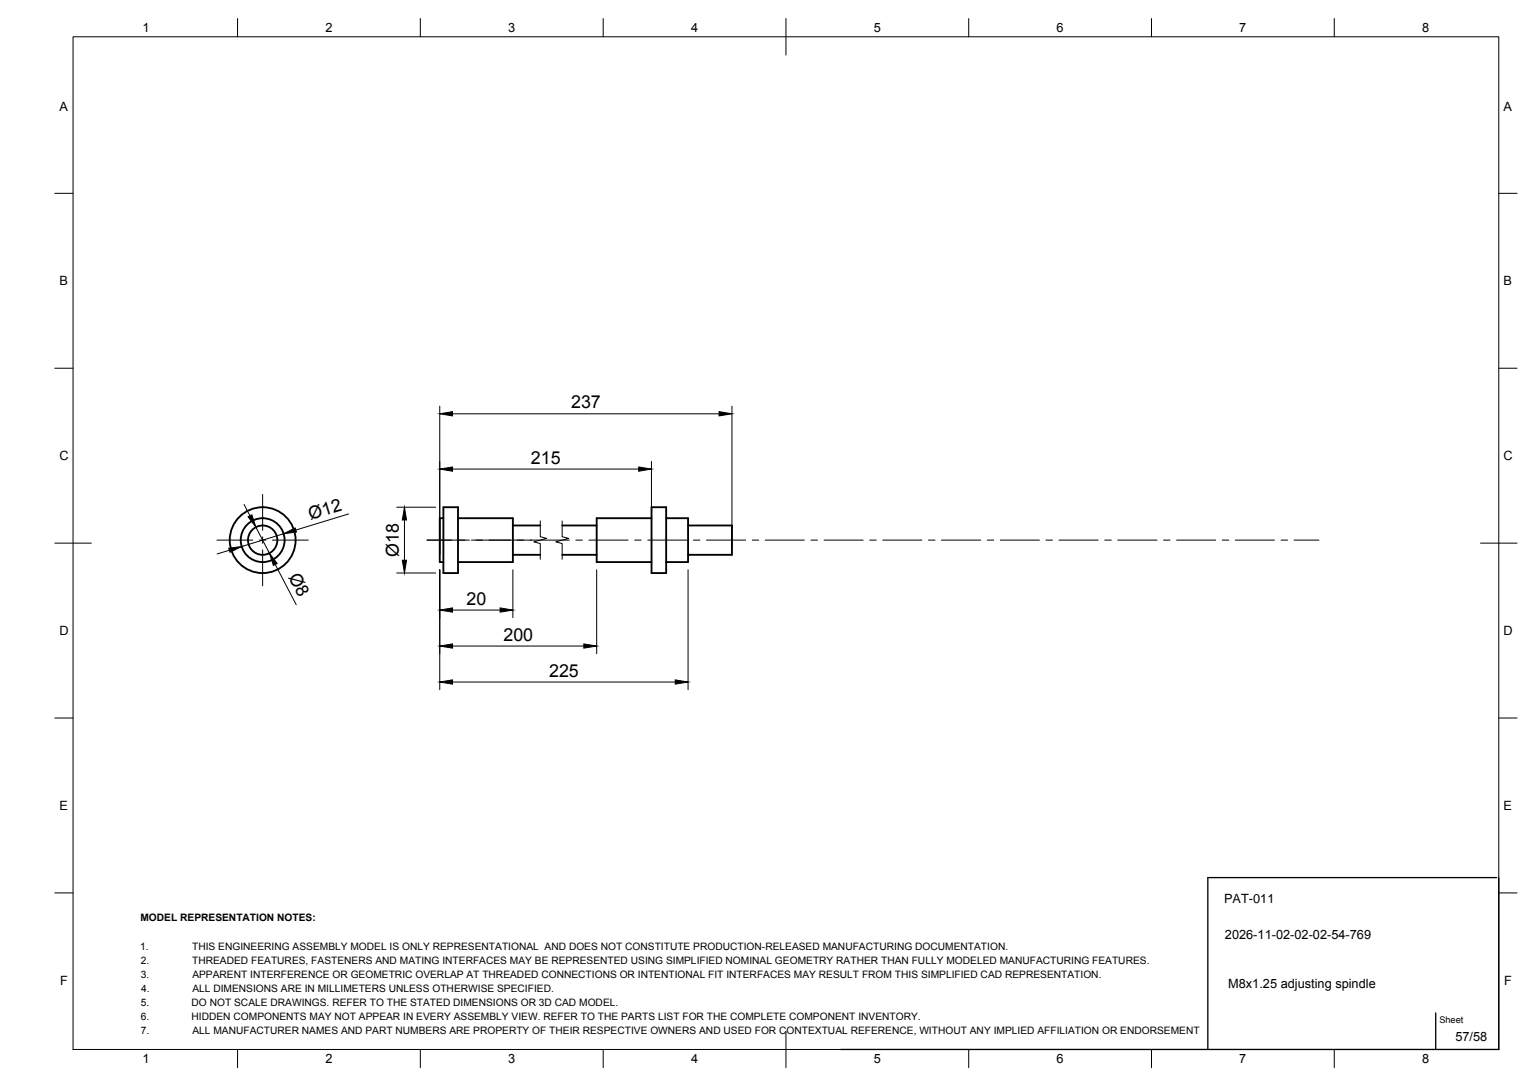
ISO-10303-21;
HEADER;
/* Generated by software containing ST-Developer
 * from STEP Tools, Inc. (www.steptools.com) 
 */

FILE_DESCRIPTION(
/* description */ ('Belt tension measurement rig'),
/* implementation_level */ '2;1');

FILE_NAME(
/* name */ 'M8x1.25 adjusting spindle.step',
/* time_stamp */ '2026-10-28T03:24:44-07:00',
/* author */ (''),
/* organization */ (''),
/* preprocessor_version */ 'ST-DEVELOPER v20.2',
/* originating_system */ 'Autodesk Translation Framework v15.17.0.0',
/* authorisation */ '');

FILE_SCHEMA (('AUTOMOTIVE_DESIGN { 1 0 10303 214 3 1 1 }'));
ENDSEC;

DATA;
#10=MECHANICAL_DESIGN_GEOMETRIC_PRESENTATION_REPRESENTATION('',(#759),#23587);
#634=SHAPE_REPRESENTATION_RELATIONSHIP('SRR','None',#23886,#689);
#689=ADVANCED_BREP_SHAPE_REPRESENTATION('',(#826),#23584);
#759=STYLED_ITEM('',(#24197),#826);
#826=MANIFOLD_SOLID_BREP('Body1',#12267);
#1027=FACE_BOUND('',#2925,.T.);
#1028=FACE_BOUND('',#2927,.T.);
#1029=FACE_BOUND('',#2931,.T.);
#1030=FACE_BOUND('',#2933,.T.);
#1031=FACE_BOUND('',#2937,.T.);
#1032=FACE_BOUND('',#2940,.T.);
#1033=FACE_BOUND('',#2945,.T.);
#1330=PLANE('',#14418);
#1331=PLANE('',#14419);
#1332=PLANE('',#14422);
#1333=PLANE('',#14428);
#1334=PLANE('',#14431);
#1335=PLANE('',#14437);
#1336=PLANE('',#14441);
#1337=PLANE('',#14446);
#1338=PLANE('',#14447);
#2020=FACE_OUTER_BOUND('',#2922,.T.);
#2021=FACE_OUTER_BOUND('',#2923,.T.);
#2022=FACE_OUTER_BOUND('',#2924,.T.);
#2023=FACE_OUTER_BOUND('',#2926,.T.);
#2024=FACE_OUTER_BOUND('',#2928,.T.);
#2025=FACE_OUTER_BOUND('',#2929,.T.);
#2026=FACE_OUTER_BOUND('',#2930,.T.);
#2027=FACE_OUTER_BOUND('',#2932,.T.);
#2028=FACE_OUTER_BOUND('',#2934,.T.);
#2029=FACE_OUTER_BOUND('',#2935,.T.);
#2030=FACE_OUTER_BOUND('',#2936,.T.);
#2031=FACE_OUTER_BOUND('',#2938,.T.);
#2032=FACE_OUTER_BOUND('',#2939,.T.);
#2033=FACE_OUTER_BOUND('',#2941,.T.);
#2034=FACE_OUTER_BOUND('',#2942,.T.);
#2035=FACE_OUTER_BOUND('',#2943,.T.);
#2036=FACE_OUTER_BOUND('',#2944,.T.);
#2922=EDGE_LOOP('',(#11020,#11021,#11022,#11023));
#2923=EDGE_LOOP('',(#11024));
#2924=EDGE_LOOP('',(#11025));
#2925=EDGE_LOOP('',(#11026));
#2926=EDGE_LOOP('',(#11027));
#2927=EDGE_LOOP('',(#11028));
#2928=EDGE_LOOP('',(#11029,#11030,#11031,#11032));
#2929=EDGE_LOOP('',(#11033,#11034,#11035,#11036));
#2930=EDGE_LOOP('',(#11037));
#2931=EDGE_LOOP('',(#11038));
#2932=EDGE_LOOP('',(#11039));
#2933=EDGE_LOOP('',(#11040));
#2934=EDGE_LOOP('',(#11041,#11042,#11043,#11044));
#2935=EDGE_LOOP('',(#11045,#11046,#11047,#11048));
#2936=EDGE_LOOP('',(#11049));
#2937=EDGE_LOOP('',(#11050));
#2938=EDGE_LOOP('',(#11051,#11052,#11053,#11054));
#2939=EDGE_LOOP('',(#11055));
#2940=EDGE_LOOP('',(#11056));
#2941=EDGE_LOOP('',(#11057,#11058,#11059,#11060));
#2942=EDGE_LOOP('',(#11061,#11062,#11063,#11064));
#2943=EDGE_LOOP('',(#11065));
#2944=EDGE_LOOP('',(#11066));
#2945=EDGE_LOOP('',(#11067));
#3683=LINE('',#23217,#4434);
#3684=LINE('',#23231,#4435);
#3685=LINE('',#23234,#4436);
#3686=LINE('',#23247,#4437);
#3687=LINE('',#23250,#4438);
#3688=LINE('',#23258,#4439);
#3689=LINE('',#23265,#4440);
#3690=LINE('',#23267,#4441);
#4434=VECTOR('',#18314,0.4);
#4435=VECTOR('',#18333,0.9);
#4436=VECTOR('',#18336,0.6);
#4437=VECTOR('',#18353,0.9);
#4438=VECTOR('',#18356,0.6);
#4439=VECTOR('',#18367,0.6);
#4440=VECTOR('',#18376,0.6);
#4441=VECTOR('',#18379,0.4);
#5212=CIRCLE('',#14416,0.4);
#5213=CIRCLE('',#14417,0.4);
#5214=CIRCLE('',#14420,0.9);
#5215=CIRCLE('',#14421,0.6);
#5216=CIRCLE('',#14423,0.9);
#5217=CIRCLE('',#14424,0.6);
#5218=CIRCLE('',#14427,0.6);
#5219=CIRCLE('',#14429,0.9);
#5220=CIRCLE('',#14430,0.6);
#5221=CIRCLE('',#14432,0.9);
#5222=CIRCLE('',#14433,0.6);
#5223=CIRCLE('',#14436,0.6);
#5224=CIRCLE('',#14438,0.4);
#5225=CIRCLE('',#14440,0.6);
#5226=CIRCLE('',#14442,0.6);
#5227=CIRCLE('',#14443,0.4);
#6283=VERTEX_POINT('',#23214);
#6284=VERTEX_POINT('',#23216);
#6285=VERTEX_POINT('',#23221);
#6286=VERTEX_POINT('',#23223);
#6287=VERTEX_POINT('',#23226);
#6288=VERTEX_POINT('',#23228);
#6289=VERTEX_POINT('',#23233);
#6290=VERTEX_POINT('',#23237);
#6291=VERTEX_POINT('',#23239);
#6292=VERTEX_POINT('',#23242);
#6293=VERTEX_POINT('',#23244);
#6294=VERTEX_POINT('',#23249);
#6295=VERTEX_POINT('',#23253);
#6296=VERTEX_POINT('',#23256);
#6297=VERTEX_POINT('',#23260);
#6298=VERTEX_POINT('',#23262);
#7869=EDGE_CURVE('',#6283,#6283,#5212,.T.);
#7870=EDGE_CURVE('',#6283,#6284,#3683,.T.);
#7871=EDGE_CURVE('',#6284,#6284,#5213,.T.);
#7872=EDGE_CURVE('',#6285,#6285,#5214,.T.);
#7873=EDGE_CURVE('',#6286,#6286,#5215,.T.);
#7874=EDGE_CURVE('',#6287,#6287,#5216,.T.);
#7875=EDGE_CURVE('',#6288,#6288,#5217,.T.);
#7876=EDGE_CURVE('',#6285,#6287,#3684,.T.);
#7877=EDGE_CURVE('',#6288,#6289,#3685,.T.);
#7878=EDGE_CURVE('',#6289,#6289,#5218,.T.);
#7879=EDGE_CURVE('',#6290,#6290,#5219,.T.);
#7880=EDGE_CURVE('',#6291,#6291,#5220,.T.);
#7881=EDGE_CURVE('',#6292,#6292,#5221,.T.);
#7882=EDGE_CURVE('',#6293,#6293,#5222,.T.);
#7883=EDGE_CURVE('',#6290,#6292,#3686,.T.);
#7884=EDGE_CURVE('',#6293,#6294,#3687,.T.);
#7885=EDGE_CURVE('',#6294,#6294,#5223,.T.);
#7886=EDGE_CURVE('',#6295,#6295,#5224,.T.);
#7887=EDGE_CURVE('',#6296,#6296,#5225,.T.);
#7888=EDGE_CURVE('',#6296,#6286,#3688,.T.);
#7889=EDGE_CURVE('',#6297,#6297,#5226,.T.);
#7890=EDGE_CURVE('',#6298,#6298,#5227,.T.);
#7891=EDGE_CURVE('',#6297,#6291,#3689,.T.);
#7892=EDGE_CURVE('',#6295,#6298,#3690,.T.);
#11020=ORIENTED_EDGE('',*,*,#7869,.F.);
#11021=ORIENTED_EDGE('',*,*,#7870,.T.);
#11022=ORIENTED_EDGE('',*,*,#7871,.T.);
#11023=ORIENTED_EDGE('',*,*,#7870,.F.);
#11024=ORIENTED_EDGE('',*,*,#7871,.F.);
#11025=ORIENTED_EDGE('',*,*,#7872,.T.);
#11026=ORIENTED_EDGE('',*,*,#7873,.F.);
#11027=ORIENTED_EDGE('',*,*,#7874,.F.);
#11028=ORIENTED_EDGE('',*,*,#7875,.F.);
#11029=ORIENTED_EDGE('',*,*,#7872,.F.);
#11030=ORIENTED_EDGE('',*,*,#7876,.T.);
#11031=ORIENTED_EDGE('',*,*,#7874,.T.);
#11032=ORIENTED_EDGE('',*,*,#7876,.F.);
#11033=ORIENTED_EDGE('',*,*,#7875,.T.);
#11034=ORIENTED_EDGE('',*,*,#7877,.T.);
#11035=ORIENTED_EDGE('',*,*,#7878,.T.);
#11036=ORIENTED_EDGE('',*,*,#7877,.F.);
#11037=ORIENTED_EDGE('',*,*,#7879,.T.);
#11038=ORIENTED_EDGE('',*,*,#7880,.F.);
#11039=ORIENTED_EDGE('',*,*,#7881,.F.);
#11040=ORIENTED_EDGE('',*,*,#7882,.F.);
#11041=ORIENTED_EDGE('',*,*,#7879,.F.);
#11042=ORIENTED_EDGE('',*,*,#7883,.T.);
#11043=ORIENTED_EDGE('',*,*,#7881,.T.);
#11044=ORIENTED_EDGE('',*,*,#7883,.F.);
#11045=ORIENTED_EDGE('',*,*,#7882,.T.);
#11046=ORIENTED_EDGE('',*,*,#7884,.T.);
#11047=ORIENTED_EDGE('',*,*,#7885,.T.);
#11048=ORIENTED_EDGE('',*,*,#7884,.F.);
#11049=ORIENTED_EDGE('',*,*,#7878,.F.);
#11050=ORIENTED_EDGE('',*,*,#7886,.F.);
#11051=ORIENTED_EDGE('',*,*,#7887,.F.);
#11052=ORIENTED_EDGE('',*,*,#7888,.T.);
#11053=ORIENTED_EDGE('',*,*,#7873,.T.);
#11054=ORIENTED_EDGE('',*,*,#7888,.F.);
#11055=ORIENTED_EDGE('',*,*,#7889,.T.);
#11056=ORIENTED_EDGE('',*,*,#7890,.F.);
#11057=ORIENTED_EDGE('',*,*,#7889,.F.);
#11058=ORIENTED_EDGE('',*,*,#7891,.T.);
#11059=ORIENTED_EDGE('',*,*,#7880,.T.);
#11060=ORIENTED_EDGE('',*,*,#7891,.F.);
#11061=ORIENTED_EDGE('',*,*,#7886,.T.);
#11062=ORIENTED_EDGE('',*,*,#7892,.T.);
#11063=ORIENTED_EDGE('',*,*,#7890,.T.);
#11064=ORIENTED_EDGE('',*,*,#7892,.F.);
#11065=ORIENTED_EDGE('',*,*,#7887,.T.);
#11066=ORIENTED_EDGE('',*,*,#7885,.F.);
#11067=ORIENTED_EDGE('',*,*,#7869,.T.);
#11481=CYLINDRICAL_SURFACE('',#14415,0.4);
#11482=CYLINDRICAL_SURFACE('',#14425,0.9);
#11483=CYLINDRICAL_SURFACE('',#14426,0.6);
#11484=CYLINDRICAL_SURFACE('',#14434,0.9);
#11485=CYLINDRICAL_SURFACE('',#14435,0.6);
#11486=CYLINDRICAL_SURFACE('',#14439,0.6);
#11487=CYLINDRICAL_SURFACE('',#14444,0.6);
#11488=CYLINDRICAL_SURFACE('',#14445,0.4);
#12161=ADVANCED_FACE('',(#2020),#11481,.T.);
#12162=ADVANCED_FACE('',(#2021),#1330,.F.);
#12163=ADVANCED_FACE('',(#2022,#1027),#1331,.T.);
#12164=ADVANCED_FACE('',(#2023,#1028),#1332,.F.);
#12165=ADVANCED_FACE('',(#2024),#11482,.T.);
#12166=ADVANCED_FACE('',(#2025),#11483,.T.);
#12167=ADVANCED_FACE('',(#2026,#1029),#1333,.T.);
#12168=ADVANCED_FACE('',(#2027,#1030),#1334,.F.);
#12169=ADVANCED_FACE('',(#2028),#11484,.T.);
#12170=ADVANCED_FACE('',(#2029),#11485,.T.);
#12171=ADVANCED_FACE('',(#2030,#1031),#1335,.F.);
#12172=ADVANCED_FACE('',(#2031),#11486,.T.);
#12173=ADVANCED_FACE('',(#2032,#1032),#1336,.T.);
#12174=ADVANCED_FACE('',(#2033),#11487,.T.);
#12175=ADVANCED_FACE('',(#2034),#11488,.T.);
#12176=ADVANCED_FACE('',(#2035),#1337,.T.);
#12177=ADVANCED_FACE('',(#2036,#1033),#1338,.F.);
#12267=CLOSED_SHELL('',(#12161,#12162,#12163,#12164,#12165,#12166,#12167,
#12168,#12169,#12170,#12171,#12172,#12173,#12174,#12175,#12176,#12177));
#14414=AXIS2_PLACEMENT_3D('',#23212,#18308,#18309);
#14415=AXIS2_PLACEMENT_3D('',#23213,#18310,#18311);
#14416=AXIS2_PLACEMENT_3D('',#23215,#18312,#18313);
#14417=AXIS2_PLACEMENT_3D('',#23218,#18315,#18316);
#14418=AXIS2_PLACEMENT_3D('',#23219,#18317,#18318);
#14419=AXIS2_PLACEMENT_3D('',#23220,#18319,#18320);
#14420=AXIS2_PLACEMENT_3D('',#23222,#18321,#18322);
#14421=AXIS2_PLACEMENT_3D('',#23224,#18323,#18324);
#14422=AXIS2_PLACEMENT_3D('',#23225,#18325,#18326);
#14423=AXIS2_PLACEMENT_3D('',#23227,#18327,#18328);
#14424=AXIS2_PLACEMENT_3D('',#23229,#18329,#18330);
#14425=AXIS2_PLACEMENT_3D('',#23230,#18331,#18332);
#14426=AXIS2_PLACEMENT_3D('',#23232,#18334,#18335);
#14427=AXIS2_PLACEMENT_3D('',#23235,#18337,#18338);
#14428=AXIS2_PLACEMENT_3D('',#23236,#18339,#18340);
#14429=AXIS2_PLACEMENT_3D('',#23238,#18341,#18342);
#14430=AXIS2_PLACEMENT_3D('',#23240,#18343,#18344);
#14431=AXIS2_PLACEMENT_3D('',#23241,#18345,#18346);
#14432=AXIS2_PLACEMENT_3D('',#23243,#18347,#18348);
#14433=AXIS2_PLACEMENT_3D('',#23245,#18349,#18350);
#14434=AXIS2_PLACEMENT_3D('',#23246,#18351,#18352);
#14435=AXIS2_PLACEMENT_3D('',#23248,#18354,#18355);
#14436=AXIS2_PLACEMENT_3D('',#23251,#18357,#18358);
#14437=AXIS2_PLACEMENT_3D('',#23252,#18359,#18360);
#14438=AXIS2_PLACEMENT_3D('',#23254,#18361,#18362);
#14439=AXIS2_PLACEMENT_3D('',#23255,#18363,#18364);
#14440=AXIS2_PLACEMENT_3D('',#23257,#18365,#18366);
#14441=AXIS2_PLACEMENT_3D('',#23259,#18368,#18369);
#14442=AXIS2_PLACEMENT_3D('',#23261,#18370,#18371);
#14443=AXIS2_PLACEMENT_3D('',#23263,#18372,#18373);
#14444=AXIS2_PLACEMENT_3D('',#23264,#18374,#18375);
#14445=AXIS2_PLACEMENT_3D('',#23266,#18377,#18378);
#14446=AXIS2_PLACEMENT_3D('',#23268,#18380,#18381);
#14447=AXIS2_PLACEMENT_3D('',#23269,#18382,#18383);
#18308=DIRECTION('axis',(0.,0.,1.));
#18309=DIRECTION('refdir',(1.,0.,0.));
#18310=DIRECTION('center_axis',(1.,0.,0.));
#18311=DIRECTION('ref_axis',(0.,0.,-1.));
#18312=DIRECTION('center_axis',(1.,0.,0.));
#18313=DIRECTION('ref_axis',(0.,0.,-1.));
#18314=DIRECTION('',(-1.,0.,0.));
#18315=DIRECTION('center_axis',(1.,0.,0.));
#18316=DIRECTION('ref_axis',(0.,0.,-1.));
#18317=DIRECTION('center_axis',(1.,0.,0.));
#18318=DIRECTION('ref_axis',(0.,0.,-1.));
#18319=DIRECTION('center_axis',(1.,0.,0.));
#18320=DIRECTION('ref_axis',(0.,0.,-1.));
#18321=DIRECTION('center_axis',(1.,0.,0.));
#18322=DIRECTION('ref_axis',(0.,0.,-1.));
#18323=DIRECTION('center_axis',(1.,0.,0.));
#18324=DIRECTION('ref_axis',(0.,0.,-1.));
#18325=DIRECTION('center_axis',(1.,0.,0.));
#18326=DIRECTION('ref_axis',(0.,0.,-1.));
#18327=DIRECTION('center_axis',(1.,0.,0.));
#18328=DIRECTION('ref_axis',(0.,0.,-1.));
#18329=DIRECTION('center_axis',(-1.,0.,0.));
#18330=DIRECTION('ref_axis',(0.,0.,-1.));
#18331=DIRECTION('center_axis',(1.,0.,0.));
#18332=DIRECTION('ref_axis',(0.,0.,-1.));
#18333=DIRECTION('',(-1.,0.,0.));
#18334=DIRECTION('center_axis',(1.,0.,0.));
#18335=DIRECTION('ref_axis',(0.,0.,-1.));
#18336=DIRECTION('',(-1.,0.,0.));
#18337=DIRECTION('center_axis',(1.,0.,0.));
#18338=DIRECTION('ref_axis',(0.,0.,-1.));
#18339=DIRECTION('center_axis',(1.,0.,0.));
#18340=DIRECTION('ref_axis',(0.,0.,-1.));
#18341=DIRECTION('center_axis',(1.,0.,0.));
#18342=DIRECTION('ref_axis',(0.,0.,-1.));
#18343=DIRECTION('center_axis',(1.,0.,0.));
#18344=DIRECTION('ref_axis',(0.,0.,-1.));
#18345=DIRECTION('center_axis',(1.,0.,0.));
#18346=DIRECTION('ref_axis',(0.,0.,-1.));
#18347=DIRECTION('center_axis',(1.,0.,0.));
#18348=DIRECTION('ref_axis',(0.,0.,-1.));
#18349=DIRECTION('center_axis',(-1.,0.,0.));
#18350=DIRECTION('ref_axis',(0.,0.,-1.));
#18351=DIRECTION('center_axis',(1.,0.,0.));
#18352=DIRECTION('ref_axis',(0.,0.,-1.));
#18353=DIRECTION('',(-1.,0.,0.));
#18354=DIRECTION('center_axis',(1.,0.,0.));
#18355=DIRECTION('ref_axis',(0.,0.,-1.));
#18356=DIRECTION('',(-1.,0.,0.));
#18357=DIRECTION('center_axis',(1.,0.,0.));
#18358=DIRECTION('ref_axis',(0.,0.,-1.));
#18359=DIRECTION('center_axis',(1.,0.,0.));
#18360=DIRECTION('ref_axis',(0.,0.,-1.));
#18361=DIRECTION('center_axis',(-1.,0.,0.));
#18362=DIRECTION('ref_axis',(0.,0.,-1.));
#18363=DIRECTION('center_axis',(1.,0.,0.));
#18364=DIRECTION('ref_axis',(0.,0.,-1.));
#18365=DIRECTION('center_axis',(1.,0.,0.));
#18366=DIRECTION('ref_axis',(0.,0.,-1.));
#18367=DIRECTION('',(-1.,0.,0.));
#18368=DIRECTION('center_axis',(1.,0.,0.));
#18369=DIRECTION('ref_axis',(0.,0.,-1.));
#18370=DIRECTION('center_axis',(1.,0.,0.));
#18371=DIRECTION('ref_axis',(0.,0.,-1.));
#18372=DIRECTION('center_axis',(1.,0.,0.));
#18373=DIRECTION('ref_axis',(0.,0.,-1.));
#18374=DIRECTION('center_axis',(1.,0.,0.));
#18375=DIRECTION('ref_axis',(0.,0.,-1.));
#18376=DIRECTION('',(-1.,0.,0.));
#18377=DIRECTION('center_axis',(1.,0.,0.));
#18378=DIRECTION('ref_axis',(0.,0.,-1.));
#18379=DIRECTION('',(-1.,0.,0.));
#18380=DIRECTION('center_axis',(1.,0.,0.));
#18381=DIRECTION('ref_axis',(0.,0.,-1.));
#18382=DIRECTION('center_axis',(1.,0.,0.));
#18383=DIRECTION('ref_axis',(0.,0.,-1.));
#23212=CARTESIAN_POINT('',(0.,0.,0.));
#23213=CARTESIAN_POINT('Origin',(-0.2,11.,4.5));
#23214=CARTESIAN_POINT('',(1.,11.,4.9));
#23215=CARTESIAN_POINT('Origin',(1.,11.,4.5));
#23216=CARTESIAN_POINT('',(-0.2,11.,4.9));
#23217=CARTESIAN_POINT('',(-0.2,11.,4.9));
#23218=CARTESIAN_POINT('Origin',(-0.2,11.,4.5));
#23219=CARTESIAN_POINT('Origin',(-0.2,11.,4.5));
#23220=CARTESIAN_POINT('Origin',(23.4,11.,4.5));
#23221=CARTESIAN_POINT('',(23.4,11.,5.4));
#23222=CARTESIAN_POINT('Origin',(23.4,11.,4.5));
#23223=CARTESIAN_POINT('',(23.4,11.,5.1));
#23224=CARTESIAN_POINT('Origin',(23.4,11.,4.5));
#23225=CARTESIAN_POINT('Origin',(23.,11.,4.5));
#23226=CARTESIAN_POINT('',(23.,11.,5.4));
#23227=CARTESIAN_POINT('Origin',(23.,11.,4.5));
#23228=CARTESIAN_POINT('',(23.,11.,5.1));
#23229=CARTESIAN_POINT('Origin',(23.,11.,4.5));
#23230=CARTESIAN_POINT('Origin',(23.,11.,4.5));
#23231=CARTESIAN_POINT('',(23.,11.,5.4));
#23232=CARTESIAN_POINT('Origin',(21.5,11.,4.5));
#23233=CARTESIAN_POINT('',(21.5,11.,5.1));
#23234=CARTESIAN_POINT('',(21.5,11.,5.1));
#23235=CARTESIAN_POINT('Origin',(21.5,11.,4.5));
#23236=CARTESIAN_POINT('Origin',(2.,11.,4.5));
#23237=CARTESIAN_POINT('',(2.,11.,5.4));
#23238=CARTESIAN_POINT('Origin',(2.,11.,4.5));
#23239=CARTESIAN_POINT('',(2.,11.,5.1));
#23240=CARTESIAN_POINT('Origin',(2.,11.,4.5));
#23241=CARTESIAN_POINT('Origin',(1.6,11.,4.5));
#23242=CARTESIAN_POINT('',(1.6,11.,5.4));
#23243=CARTESIAN_POINT('Origin',(1.6,11.,4.5));
#23244=CARTESIAN_POINT('',(1.6,11.,5.1));
#23245=CARTESIAN_POINT('Origin',(1.6,11.,4.5));
#23246=CARTESIAN_POINT('Origin',(1.6,11.,4.5));
#23247=CARTESIAN_POINT('',(1.6,11.,5.4));
#23248=CARTESIAN_POINT('Origin',(1.,11.,4.5));
#23249=CARTESIAN_POINT('',(1.,11.,5.1));
#23250=CARTESIAN_POINT('',(1.,11.,5.1));
#23251=CARTESIAN_POINT('Origin',(1.,11.,4.5));
#23252=CARTESIAN_POINT('Origin',(21.5,11.,4.5));
#23253=CARTESIAN_POINT('',(21.5,11.,4.9));
#23254=CARTESIAN_POINT('Origin',(21.5,11.,4.5));
#23255=CARTESIAN_POINT('Origin',(21.5,11.,4.5));
#23256=CARTESIAN_POINT('',(23.5,11.,5.1));
#23257=CARTESIAN_POINT('Origin',(23.5,11.,4.5));
#23258=CARTESIAN_POINT('',(21.5,11.,5.1));
#23259=CARTESIAN_POINT('Origin',(3.5,11.,4.5));
#23260=CARTESIAN_POINT('',(3.5,11.,5.1));
#23261=CARTESIAN_POINT('Origin',(3.5,11.,4.5));
#23262=CARTESIAN_POINT('',(3.5,11.,4.9));
#23263=CARTESIAN_POINT('Origin',(3.5,11.,4.5));
#23264=CARTESIAN_POINT('Origin',(1.,11.,4.5));
#23265=CARTESIAN_POINT('',(1.,11.,5.1));
#23266=CARTESIAN_POINT('Origin',(1.,11.,4.5));
#23267=CARTESIAN_POINT('',(1.,11.,4.9));
#23268=CARTESIAN_POINT('Origin',(23.5,11.,4.5));
#23269=CARTESIAN_POINT('Origin',(1.,11.,4.5));
#23519=UNCERTAINTY_MEASURE_WITH_UNIT(LENGTH_MEASURE(0.001),#23588,
'DISTANCE_ACCURACY_VALUE',
'Maximum model space distance between geometric entities at asserted c
onnectivities');
#23522=UNCERTAINTY_MEASURE_WITH_UNIT(LENGTH_MEASURE(0.001),#23588,
'DISTANCE_ACCURACY_VALUE',
'Maximum model space distance between geometric entities at asserted c
onnectivities');
#23584=(
GEOMETRIC_REPRESENTATION_CONTEXT(3)
GLOBAL_UNCERTAINTY_ASSIGNED_CONTEXT((#23519))
GLOBAL_UNIT_ASSIGNED_CONTEXT((#23588,#23590,#23591))
REPRESENTATION_CONTEXT('','3D')
);
#23587=(
GEOMETRIC_REPRESENTATION_CONTEXT(3)
GLOBAL_UNCERTAINTY_ASSIGNED_CONTEXT((#23522))
GLOBAL_UNIT_ASSIGNED_CONTEXT((#23588,#23590,#23591))
REPRESENTATION_CONTEXT('','3D')
);
#23588=(
LENGTH_UNIT()
NAMED_UNIT(*)
SI_UNIT(.CENTI.,.METRE.)
);
#23590=(
NAMED_UNIT(*)
PLANE_ANGLE_UNIT()
SI_UNIT($,.RADIAN.)
);
#23591=(
NAMED_UNIT(*)
SI_UNIT($,.STERADIAN.)
SOLID_ANGLE_UNIT()
);
#23653=SHAPE_DEFINITION_REPRESENTATION(#23784,#23886);
#23784=PRODUCT_DEFINITION_SHAPE('',$,#23951);
#23886=SHAPE_REPRESENTATION('',(#14414),#23584);
#23889=PRODUCT_DEFINITION_CONTEXT('part definition',#24083,'design');
#23951=PRODUCT_DEFINITION('M8x1.25 adjusting spindle',
'M8x1.25 adjusting spindle',#24015,#23889);
#24015=PRODUCT_DEFINITION_FORMATION('',$,#24146);
#24083=APPLICATION_CONTEXT(
'Core Data for Automotive Mechanical Design Process');
#24084=PRODUCT_CONTEXT('part definition',#24083,'mechanical');
#24146=PRODUCT('M8x1.25 adjusting spindle','M8x1.25 adjusting spindle',
'M8x1.25 adjusting spindle',(#24084));
#24191=COLOUR_RGB('Light Blue',0.38,0.62,0.78);
#24192=FILL_AREA_STYLE_COLOUR('',#24191);
#24193=FILL_AREA_STYLE('',(#24192));
#24194=SURFACE_STYLE_FILL_AREA(#24193);
#24195=SURFACE_SIDE_STYLE('',(#24194));
#24196=SURFACE_STYLE_USAGE(.BOTH.,#24195);
#24197=PRESENTATION_STYLE_ASSIGNMENT((#24196));
ENDSEC;
END-ISO-10303-21;
